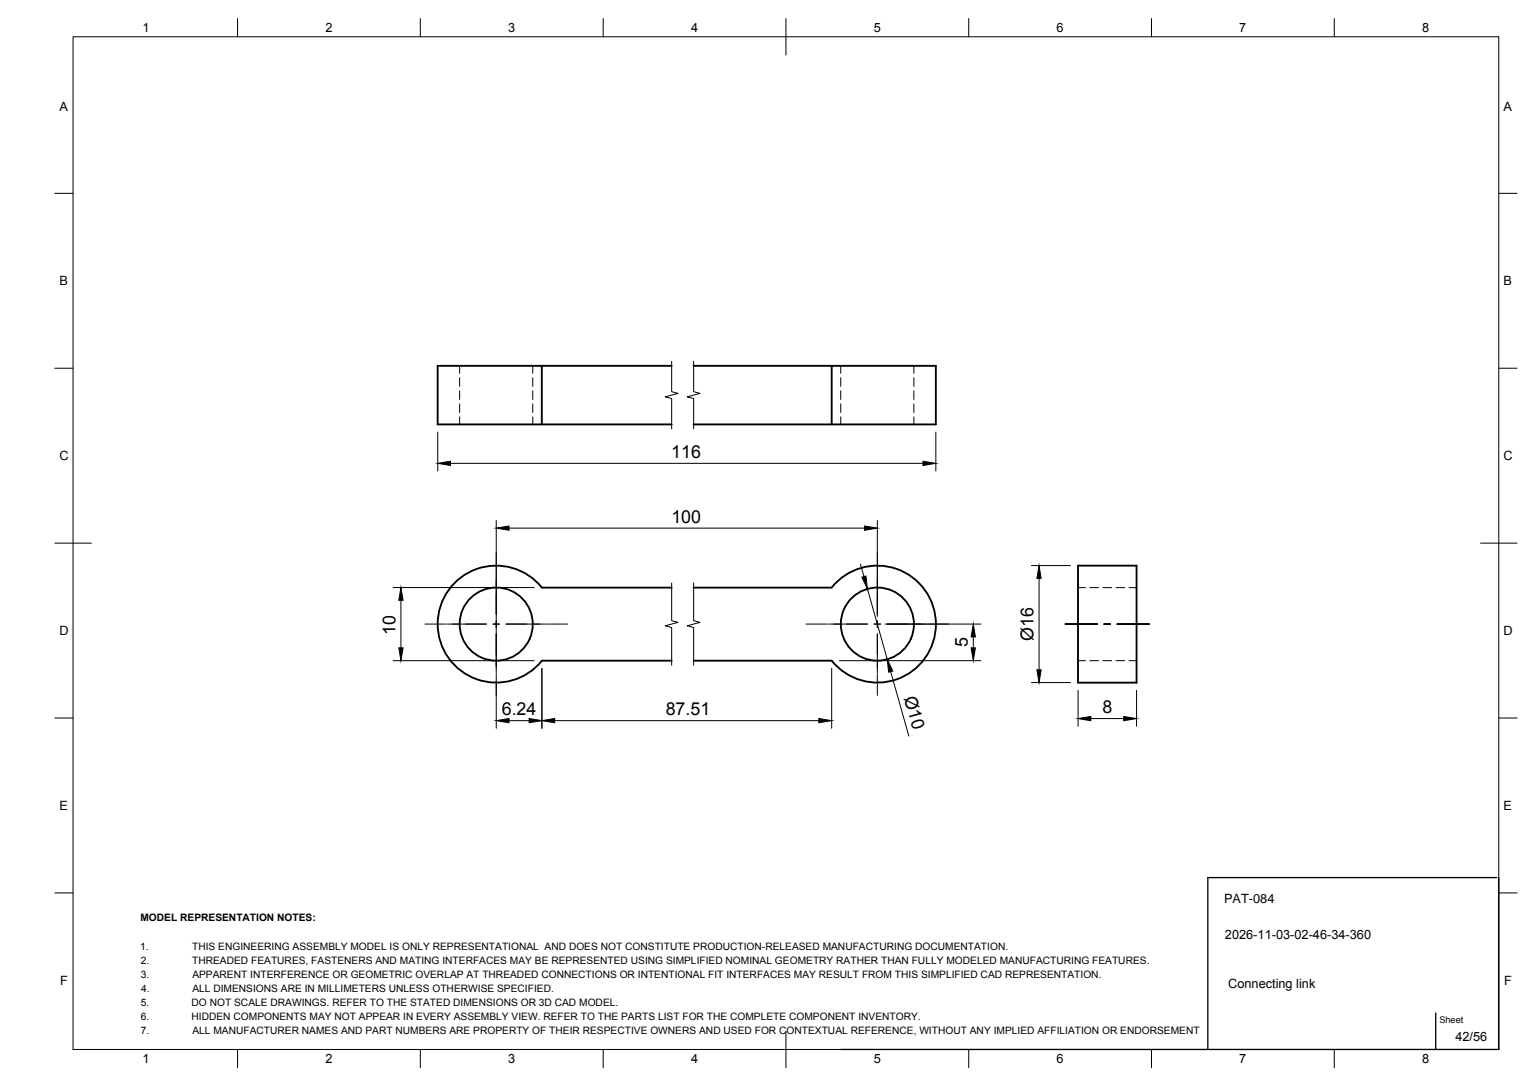
ISO-10303-21;
HEADER;
/* Generated by software containing ST-Developer
 * from STEP Tools, Inc. (www.steptools.com) 
 */

FILE_DESCRIPTION(
/* description */ ('Quick-return (Whitworth) mechanism'),
/* implementation_level */ '2;1');

FILE_NAME(
/* name */ 'Connecting link.step',
/* time_stamp */ '2026-10-28T03:25:57-07:00',
/* author */ (''),
/* organization */ (''),
/* preprocessor_version */ 'ST-DEVELOPER v20.2',
/* originating_system */ 'Autodesk Translation Framework v15.17.0.0',
/* authorisation */ '');

FILE_SCHEMA (('AUTOMOTIVE_DESIGN { 1 0 10303 214 3 1 1 }'));
ENDSEC;

DATA;
#10=MECHANICAL_DESIGN_GEOMETRIC_PRESENTATION_REPRESENTATION('',(#529),#14878);
#433=SHAPE_REPRESENTATION_RELATIONSHIP('SRR','None',#15106,#477);
#477=ADVANCED_BREP_SHAPE_REPRESENTATION('',(#580),#14863);
#529=STYLED_ITEM('',(#15399),#580);
#580=MANIFOLD_SOLID_BREP('Body1',#7884);
#749=FACE_BOUND('',#2020,.T.);
#750=FACE_BOUND('',#2021,.T.);
#751=FACE_BOUND('',#2025,.T.);
#752=FACE_BOUND('',#2026,.T.);
#962=PLANE('',#9121);
#963=PLANE('',#9122);
#964=PLANE('',#9124);
#965=PLANE('',#9127);
#1391=FACE_OUTER_BOUND('',#2015,.T.);
#1392=FACE_OUTER_BOUND('',#2016,.T.);
#1393=FACE_OUTER_BOUND('',#2017,.T.);
#1394=FACE_OUTER_BOUND('',#2018,.T.);
#1395=FACE_OUTER_BOUND('',#2019,.T.);
#1396=FACE_OUTER_BOUND('',#2022,.T.);
#1397=FACE_OUTER_BOUND('',#2023,.T.);
#1398=FACE_OUTER_BOUND('',#2024,.T.);
#2015=EDGE_LOOP('',(#6676,#6677,#6678,#6679));
#2016=EDGE_LOOP('',(#6680,#6681,#6682,#6683));
#2017=EDGE_LOOP('',(#6684,#6685,#6686,#6687));
#2018=EDGE_LOOP('',(#6688,#6689,#6690,#6691));
#2019=EDGE_LOOP('',(#6692,#6693,#6694,#6695));
#2020=EDGE_LOOP('',(#6696));
#2021=EDGE_LOOP('',(#6697));
#2022=EDGE_LOOP('',(#6698,#6699,#6700,#6701));
#2023=EDGE_LOOP('',(#6702,#6703,#6704,#6705));
#2024=EDGE_LOOP('',(#6706,#6707,#6708,#6709));
#2025=EDGE_LOOP('',(#6710));
#2026=EDGE_LOOP('',(#6711));
#2502=LINE('',#14123,#3025);
#2503=LINE('',#14129,#3026);
#2504=LINE('',#14134,#3027);
#2505=LINE('',#14138,#3028);
#2506=LINE('',#14142,#3029);
#2507=LINE('',#14144,#3030);
#2508=LINE('',#14145,#3031);
#2509=LINE('',#14148,#3032);
#2510=LINE('',#14152,#3033);
#2511=LINE('',#14153,#3034);
#3025=VECTOR('',#11189,0.5);
#3026=VECTOR('',#11196,0.5);
#3027=VECTOR('',#11201,1.);
#3028=VECTOR('',#11204,1.);
#3029=VECTOR('',#11209,1.);
#3030=VECTOR('',#11210,1.);
#3031=VECTOR('',#11211,1.);
#3032=VECTOR('',#11214,1.);
#3033=VECTOR('',#11219,1.);
#3034=VECTOR('',#11220,1.);
#3555=CIRCLE('',#9113,0.5);
#3556=CIRCLE('',#9114,0.5);
#3557=CIRCLE('',#9116,0.5);
#3558=CIRCLE('',#9117,0.5);
#3559=CIRCLE('',#9119,0.800000000000001);
#3560=CIRCLE('',#9120,0.800000000000001);
#3561=CIRCLE('',#9123,0.8);
#3562=CIRCLE('',#9126,0.8);
#4112=VERTEX_POINT('',#14120);
#4113=VERTEX_POINT('',#14122);
#4114=VERTEX_POINT('',#14126);
#4115=VERTEX_POINT('',#14128);
#4116=VERTEX_POINT('',#14132);
#4117=VERTEX_POINT('',#14133);
#4118=VERTEX_POINT('',#14135);
#4119=VERTEX_POINT('',#14137);
#4120=VERTEX_POINT('',#14141);
#4121=VERTEX_POINT('',#14143);
#4122=VERTEX_POINT('',#14147);
#4123=VERTEX_POINT('',#14151);
#4995=EDGE_CURVE('',#4112,#4112,#3555,.T.);
#4996=EDGE_CURVE('',#4112,#4113,#2502,.T.);
#4997=EDGE_CURVE('',#4113,#4113,#3556,.T.);
#4998=EDGE_CURVE('',#4114,#4114,#3557,.T.);
#4999=EDGE_CURVE('',#4114,#4115,#2503,.T.);
#5000=EDGE_CURVE('',#4115,#4115,#3558,.T.);
#5001=EDGE_CURVE('',#4116,#4117,#2504,.T.);
#5002=EDGE_CURVE('',#4118,#4116,#3559,.T.);
#5003=EDGE_CURVE('',#4119,#4118,#2505,.T.);
#5004=EDGE_CURVE('',#4119,#4117,#3560,.T.);
#5005=EDGE_CURVE('',#4120,#4117,#2506,.T.);
#5006=EDGE_CURVE('',#4121,#4120,#2507,.T.);
#5007=EDGE_CURVE('',#4116,#4121,#2508,.T.);
#5008=EDGE_CURVE('',#4119,#4122,#2509,.T.);
#5009=EDGE_CURVE('',#4120,#4122,#3561,.T.);
#5010=EDGE_CURVE('',#4123,#4118,#2510,.T.);
#5011=EDGE_CURVE('',#4122,#4123,#2511,.T.);
#5012=EDGE_CURVE('',#4121,#4123,#3562,.T.);
#6676=ORIENTED_EDGE('',*,*,#4995,.F.);
#6677=ORIENTED_EDGE('',*,*,#4996,.T.);
#6678=ORIENTED_EDGE('',*,*,#4997,.F.);
#6679=ORIENTED_EDGE('',*,*,#4996,.F.);
#6680=ORIENTED_EDGE('',*,*,#4998,.F.);
#6681=ORIENTED_EDGE('',*,*,#4999,.T.);
#6682=ORIENTED_EDGE('',*,*,#5000,.F.);
#6683=ORIENTED_EDGE('',*,*,#4999,.F.);
#6684=ORIENTED_EDGE('',*,*,#5001,.F.);
#6685=ORIENTED_EDGE('',*,*,#5002,.F.);
#6686=ORIENTED_EDGE('',*,*,#5003,.F.);
#6687=ORIENTED_EDGE('',*,*,#5004,.T.);
#6688=ORIENTED_EDGE('',*,*,#5001,.T.);
#6689=ORIENTED_EDGE('',*,*,#5005,.F.);
#6690=ORIENTED_EDGE('',*,*,#5006,.F.);
#6691=ORIENTED_EDGE('',*,*,#5007,.F.);
#6692=ORIENTED_EDGE('',*,*,#5004,.F.);
#6693=ORIENTED_EDGE('',*,*,#5008,.T.);
#6694=ORIENTED_EDGE('',*,*,#5009,.F.);
#6695=ORIENTED_EDGE('',*,*,#5005,.T.);
#6696=ORIENTED_EDGE('',*,*,#4995,.T.);
#6697=ORIENTED_EDGE('',*,*,#4998,.T.);
#6698=ORIENTED_EDGE('',*,*,#5003,.T.);
#6699=ORIENTED_EDGE('',*,*,#5010,.F.);
#6700=ORIENTED_EDGE('',*,*,#5011,.F.);
#6701=ORIENTED_EDGE('',*,*,#5008,.F.);
#6702=ORIENTED_EDGE('',*,*,#5006,.T.);
#6703=ORIENTED_EDGE('',*,*,#5009,.T.);
#6704=ORIENTED_EDGE('',*,*,#5011,.T.);
#6705=ORIENTED_EDGE('',*,*,#5012,.F.);
#6706=ORIENTED_EDGE('',*,*,#5007,.T.);
#6707=ORIENTED_EDGE('',*,*,#5012,.T.);
#6708=ORIENTED_EDGE('',*,*,#5010,.T.);
#6709=ORIENTED_EDGE('',*,*,#5002,.T.);
#6710=ORIENTED_EDGE('',*,*,#4997,.T.);
#6711=ORIENTED_EDGE('',*,*,#5000,.T.);
#7347=CYLINDRICAL_SURFACE('',#9112,0.5);
#7348=CYLINDRICAL_SURFACE('',#9115,0.5);
#7349=CYLINDRICAL_SURFACE('',#9118,0.800000000000001);
#7350=CYLINDRICAL_SURFACE('',#9125,0.8);
#7722=ADVANCED_FACE('',(#1391),#7347,.F.);
#7723=ADVANCED_FACE('',(#1392),#7348,.F.);
#7724=ADVANCED_FACE('',(#1393),#7349,.T.);
#7725=ADVANCED_FACE('',(#1394),#962,.T.);
#7726=ADVANCED_FACE('',(#1395,#749,#750),#963,.F.);
#7727=ADVANCED_FACE('',(#1396),#964,.T.);
#7728=ADVANCED_FACE('',(#1397),#7350,.T.);
#7729=ADVANCED_FACE('',(#1398,#751,#752),#965,.T.);
#7884=CLOSED_SHELL('',(#7722,#7723,#7724,#7725,#7726,#7727,#7728,#7729));
#9111=AXIS2_PLACEMENT_3D('',#14118,#11183,#11184);
#9112=AXIS2_PLACEMENT_3D('',#14119,#11185,#11186);
#9113=AXIS2_PLACEMENT_3D('',#14121,#11187,#11188);
#9114=AXIS2_PLACEMENT_3D('',#14124,#11190,#11191);
#9115=AXIS2_PLACEMENT_3D('',#14125,#11192,#11193);
#9116=AXIS2_PLACEMENT_3D('',#14127,#11194,#11195);
#9117=AXIS2_PLACEMENT_3D('',#14130,#11197,#11198);
#9118=AXIS2_PLACEMENT_3D('',#14131,#11199,#11200);
#9119=AXIS2_PLACEMENT_3D('',#14136,#11202,#11203);
#9120=AXIS2_PLACEMENT_3D('',#14139,#11205,#11206);
#9121=AXIS2_PLACEMENT_3D('',#14140,#11207,#11208);
#9122=AXIS2_PLACEMENT_3D('',#14146,#11212,#11213);
#9123=AXIS2_PLACEMENT_3D('',#14149,#11215,#11216);
#9124=AXIS2_PLACEMENT_3D('',#14150,#11217,#11218);
#9125=AXIS2_PLACEMENT_3D('',#14154,#11221,#11222);
#9126=AXIS2_PLACEMENT_3D('',#14155,#11223,#11224);
#9127=AXIS2_PLACEMENT_3D('',#14156,#11225,#11226);
#11183=DIRECTION('axis',(0.,0.,1.));
#11184=DIRECTION('refdir',(1.,0.,0.));
#11185=DIRECTION('center_axis',(0.,0.,1.));
#11186=DIRECTION('ref_axis',(1.,0.,0.));
#11187=DIRECTION('center_axis',(0.,0.,1.));
#11188=DIRECTION('ref_axis',(1.,0.,0.));
#11189=DIRECTION('',(0.,0.,1.));
#11190=DIRECTION('center_axis',(0.,0.,-1.));
#11191=DIRECTION('ref_axis',(1.,0.,0.));
#11192=DIRECTION('center_axis',(0.,0.,1.));
#11193=DIRECTION('ref_axis',(1.,0.,0.));
#11194=DIRECTION('center_axis',(0.,0.,1.));
#11195=DIRECTION('ref_axis',(1.,0.,0.));
#11196=DIRECTION('',(0.,0.,1.));
#11197=DIRECTION('center_axis',(0.,0.,-1.));
#11198=DIRECTION('ref_axis',(1.,0.,0.));
#11199=DIRECTION('center_axis',(0.,0.,1.));
#11200=DIRECTION('ref_axis',(1.,0.,0.));
#11201=DIRECTION('',(0.,0.,-1.));
#11202=DIRECTION('center_axis',(0.,0.,1.));
#11203=DIRECTION('ref_axis',(1.,0.,0.));
#11204=DIRECTION('',(0.,0.,1.));
#11205=DIRECTION('center_axis',(0.,0.,1.));
#11206=DIRECTION('ref_axis',(1.,0.,0.));
#11207=DIRECTION('center_axis',(-0.4,0.916515138991168,0.));
#11208=DIRECTION('ref_axis',(-0.916515138991168,-0.4,0.));
#11209=DIRECTION('',(0.916515138991168,0.4,0.));
#11210=DIRECTION('',(0.,0.,-1.));
#11211=DIRECTION('',(-0.916515138991168,-0.4,0.));
#11212=DIRECTION('center_axis',(0.,0.,1.));
#11213=DIRECTION('ref_axis',(1.,0.,0.));
#11214=DIRECTION('',(-0.916515138991168,-0.4,0.));
#11215=DIRECTION('center_axis',(0.,0.,1.));
#11216=DIRECTION('ref_axis',(1.,0.,0.));
#11217=DIRECTION('center_axis',(0.4,-0.916515138991168,0.));
#11218=DIRECTION('ref_axis',(0.916515138991168,0.4,0.));
#11219=DIRECTION('',(0.916515138991168,0.4,0.));
#11220=DIRECTION('',(0.,0.,1.));
#11221=DIRECTION('center_axis',(0.,0.,1.));
#11222=DIRECTION('ref_axis',(-0.916515138991168,-0.4,0.));
#11223=DIRECTION('center_axis',(0.,0.,1.));
#11224=DIRECTION('ref_axis',(1.,0.,0.));
#11225=DIRECTION('center_axis',(0.,0.,1.));
#11226=DIRECTION('ref_axis',(1.,0.,0.));
#14118=CARTESIAN_POINT('',(0.,0.,0.));
#14119=CARTESIAN_POINT('Origin',(0.,12.,8.3));
#14120=CARTESIAN_POINT('',(-0.5,12.,8.4));
#14121=CARTESIAN_POINT('Origin',(0.,12.,8.4));
#14122=CARTESIAN_POINT('',(-0.5,12.,9.2));
#14123=CARTESIAN_POINT('',(-0.5,12.,8.3));
#14124=CARTESIAN_POINT('Origin',(0.,12.,9.2));
#14125=CARTESIAN_POINT('Origin',(9.16515138991168,16.,8.3));
#14126=CARTESIAN_POINT('',(8.66515138991168,16.,8.4));
#14127=CARTESIAN_POINT('Origin',(9.16515138991168,16.,8.4));
#14128=CARTESIAN_POINT('',(8.66515138991168,16.,9.2));
#14129=CARTESIAN_POINT('',(8.66515138991168,16.,8.3));
#14130=CARTESIAN_POINT('Origin',(9.16515138991168,16.,9.2));
#14131=CARTESIAN_POINT('Origin',(9.16515138991168,16.,8.4));
#14132=CARTESIAN_POINT('',(8.39278786906151,16.2084576495596,9.2));
#14133=CARTESIAN_POINT('',(8.39278786906151,16.2084576495596,8.4));
#14134=CARTESIAN_POINT('',(8.39278786906151,16.2084576495596,8.4));
#14135=CARTESIAN_POINT('',(8.79278786906151,15.2919425105685,9.2));
#14136=CARTESIAN_POINT('Origin',(9.16515138991168,16.,9.2));
#14137=CARTESIAN_POINT('',(8.79278786906151,15.2919425105685,8.4));
#14138=CARTESIAN_POINT('',(8.79278786906151,15.2919425105685,8.4));
#14139=CARTESIAN_POINT('Origin',(9.16515138991168,16.,8.4));
#14140=CARTESIAN_POINT('Origin',(8.96515138991168,16.4582575694956,8.4));
#14141=CARTESIAN_POINT('',(0.372363520850169,12.7080574894315,8.4));
#14142=CARTESIAN_POINT('',(-0.2,12.4582575694956,8.4));
#14143=CARTESIAN_POINT('',(0.372363520850169,12.7080574894315,9.2));
#14144=CARTESIAN_POINT('',(0.372363520850169,12.7080574894315,8.4));
#14145=CARTESIAN_POINT('',(-0.2,12.4582575694956,9.2));
#14146=CARTESIAN_POINT('Origin',(0.,12.,8.4));
#14147=CARTESIAN_POINT('',(0.772363520850167,11.7915423504404,8.4));
#14148=CARTESIAN_POINT('',(9.36515138991168,15.5417424305044,8.4));
#14149=CARTESIAN_POINT('Origin',(0.,12.,8.4));
#14150=CARTESIAN_POINT('Origin',(0.199999999999999,11.5417424305044,8.4));
#14151=CARTESIAN_POINT('',(0.772363520850167,11.7915423504404,9.2));
#14152=CARTESIAN_POINT('',(9.36515138991168,15.5417424305044,9.2));
#14153=CARTESIAN_POINT('',(0.772363520850168,11.7915423504404,8.4));
#14154=CARTESIAN_POINT('Origin',(0.,12.,8.4));
#14155=CARTESIAN_POINT('Origin',(0.,12.,9.2));
#14156=CARTESIAN_POINT('Origin',(0.,12.,9.2));
#14809=UNCERTAINTY_MEASURE_WITH_UNIT(LENGTH_MEASURE(0.001),#14879,
'DISTANCE_ACCURACY_VALUE',
'Maximum model space distance between geometric entities at asserted c
onnectivities');
#14824=UNCERTAINTY_MEASURE_WITH_UNIT(LENGTH_MEASURE(0.001),#14879,
'DISTANCE_ACCURACY_VALUE',
'Maximum model space distance between geometric entities at asserted c
onnectivities');
#14863=(
GEOMETRIC_REPRESENTATION_CONTEXT(3)
GLOBAL_UNCERTAINTY_ASSIGNED_CONTEXT((#14809))
GLOBAL_UNIT_ASSIGNED_CONTEXT((#14879,#14881,#14882))
REPRESENTATION_CONTEXT('','3D')
);
#14878=(
GEOMETRIC_REPRESENTATION_CONTEXT(3)
GLOBAL_UNCERTAINTY_ASSIGNED_CONTEXT((#14824))
GLOBAL_UNIT_ASSIGNED_CONTEXT((#14879,#14881,#14882))
REPRESENTATION_CONTEXT('','3D')
);
#14879=(
LENGTH_UNIT()
NAMED_UNIT(*)
SI_UNIT(.CENTI.,.METRE.)
);
#14881=(
NAMED_UNIT(*)
PLANE_ANGLE_UNIT()
SI_UNIT($,.RADIAN.)
);
#14882=(
NAMED_UNIT(*)
SI_UNIT($,.STERADIAN.)
SOLID_ANGLE_UNIT()
);
#14921=SHAPE_DEFINITION_REPRESENTATION(#14980,#15106);
#14980=PRODUCT_DEFINITION_SHAPE('',$,#15160);
#15106=SHAPE_REPRESENTATION('',(#9111),#14863);
#15121=PRODUCT_DEFINITION_CONTEXT('part definition',#15282,'design');
#15160=PRODUCT_DEFINITION('Connecting link','Connecting link',#15213,#15121);
#15213=PRODUCT_DEFINITION_FORMATION('',$,#15322);
#15282=APPLICATION_CONTEXT(
'Core Data for Automotive Mechanical Design Process');
#15283=PRODUCT_CONTEXT('part definition',#15282,'mechanical');
#15322=PRODUCT('Connecting link','Connecting link','Connecting link',(#15283));
#15393=COLOUR_RGB('Sky Blue',0.24,0.69,0.87);
#15394=FILL_AREA_STYLE_COLOUR('',#15393);
#15395=FILL_AREA_STYLE('',(#15394));
#15396=SURFACE_STYLE_FILL_AREA(#15395);
#15397=SURFACE_SIDE_STYLE('',(#15396));
#15398=SURFACE_STYLE_USAGE(.BOTH.,#15397);
#15399=PRESENTATION_STYLE_ASSIGNMENT((#15398));
ENDSEC;
END-ISO-10303-21;
